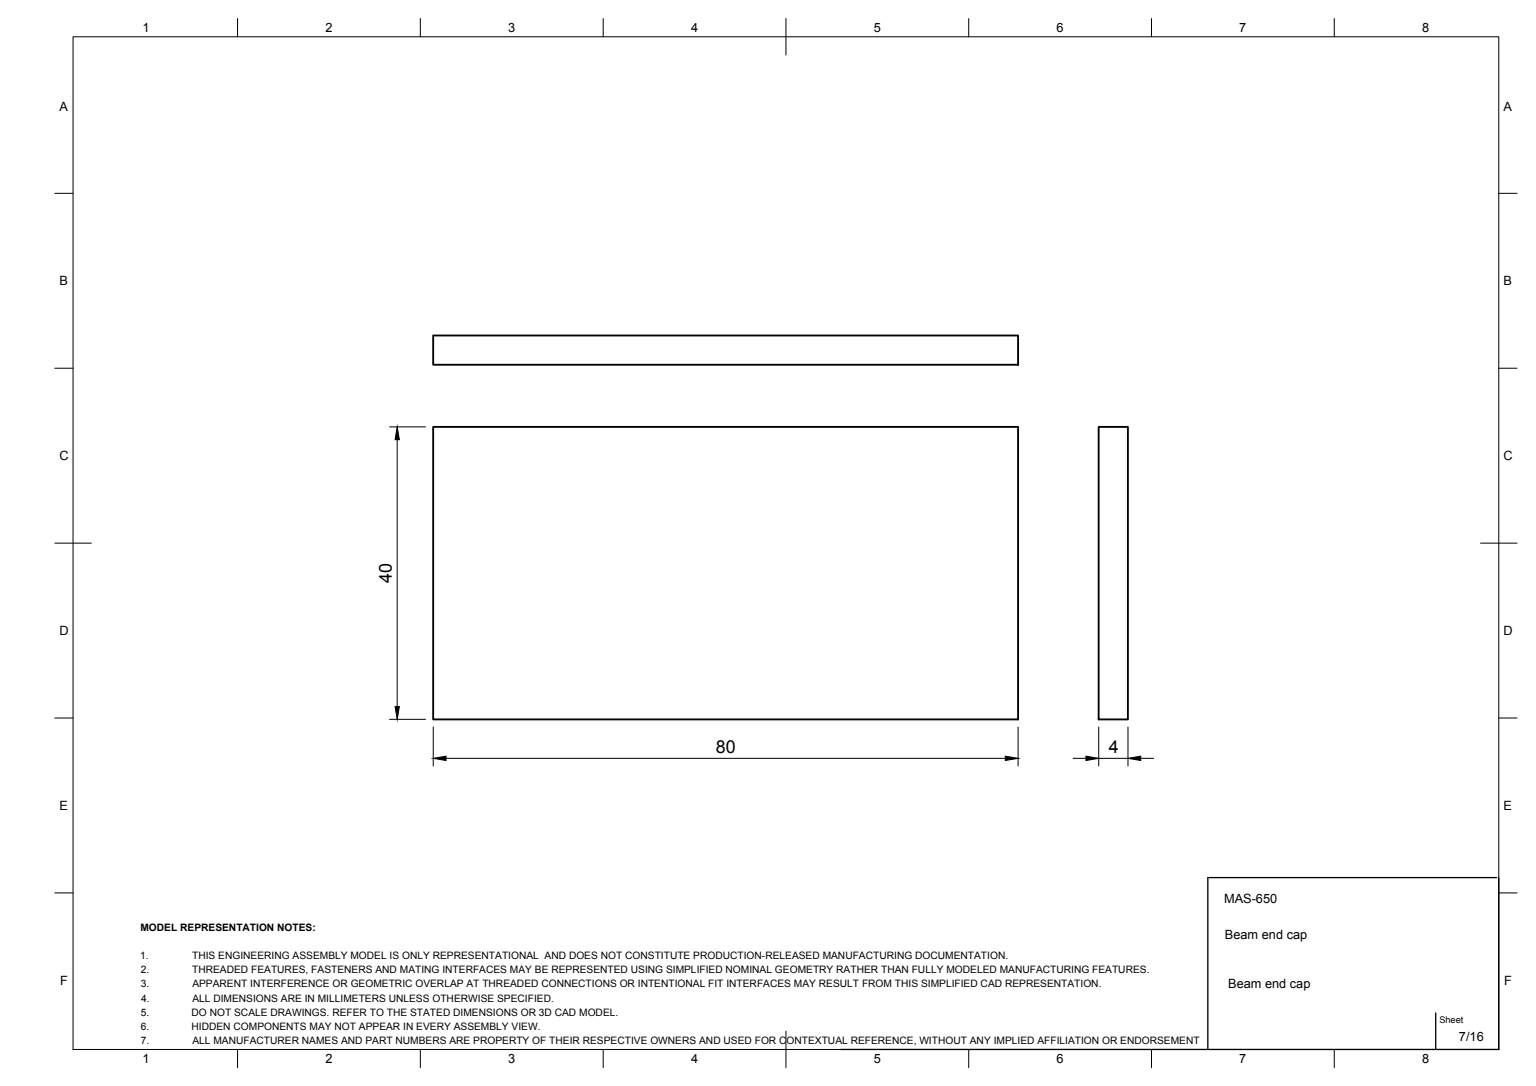
ISO-10303-21;
HEADER;
/* Generated by software containing ST-Developer
 * from STEP Tools, Inc. (www.steptools.com) 
 */

FILE_DESCRIPTION(
/* description */ ('Independent manual traversing gantry with native reusable aluminum pr
ofiles,180mm captured carriage travel, four bronze-bushed rollers, lin
ked ideal rolling motion, bonded acetal lateral guides, positive welde
d end stops and fully retained axle stacks. Editable native profile cu
t lengths220/400mm. Tool attachments viaM6 bridge-plate taps; mounted 
tool outside assembly. Welds, anchors, adhesives, fits, traction, load
/speed/structural/life ratings unassigned.'),
/* implementation_level */ '2;1');

FILE_NAME(
/* name */ 'Beam end cap.step',
/* time_stamp */ '2026-11-09T20:04:38-08:00',
/* author */ (''),
/* organization */ (''),
/* preprocessor_version */ 'ST-DEVELOPER v20.2',
/* originating_system */ 'Autodesk Translation Framework v15.17.0.0',
/* authorisation */ '');

FILE_SCHEMA (('AUTOMOTIVE_DESIGN { 1 0 10303 214 3 1 1 }'));
ENDSEC;

DATA;
#10=MECHANICAL_DESIGN_GEOMETRIC_PRESENTATION_REPRESENTATION('',(#475),#13231);
#443=SHAPE_REPRESENTATION_RELATIONSHIP('SRR','None',#13332,#459);
#459=ADVANCED_BREP_SHAPE_REPRESENTATION('',(#491),#13219);
#475=STYLED_ITEM('',(#13421),#491);
#491=MANIFOLD_SOLID_BREP('Body1',#4155);
#584=PLANE('',#4454);
#585=PLANE('',#4455);
#586=PLANE('',#4456);
#587=PLANE('',#4457);
#588=PLANE('',#4458);
#589=PLANE('',#4459);
#689=FACE_OUTER_BOUND('',#930,.T.);
#690=FACE_OUTER_BOUND('',#931,.T.);
#691=FACE_OUTER_BOUND('',#932,.T.);
#692=FACE_OUTER_BOUND('',#933,.T.);
#693=FACE_OUTER_BOUND('',#934,.T.);
#694=FACE_OUTER_BOUND('',#935,.T.);
#930=EDGE_LOOP('',(#2970,#2971,#2972,#2973));
#931=EDGE_LOOP('',(#2974,#2975,#2976,#2977));
#932=EDGE_LOOP('',(#2978,#2979,#2980,#2981));
#933=EDGE_LOOP('',(#2982,#2983,#2984,#2985));
#934=EDGE_LOOP('',(#2986,#2987,#2988,#2989));
#935=EDGE_LOOP('',(#2990,#2991,#2992,#2993));
#1220=LINE('',#6084,#1482);
#1221=LINE('',#6086,#1483);
#1222=LINE('',#6088,#1484);
#1223=LINE('',#6089,#1485);
#1224=LINE('',#6092,#1486);
#1225=LINE('',#6094,#1487);
#1226=LINE('',#6095,#1488);
#1227=LINE('',#6098,#1489);
#1228=LINE('',#6100,#1490);
#1229=LINE('',#6101,#1491);
#1230=LINE('',#6103,#1492);
#1231=LINE('',#6104,#1493);
#1482=VECTOR('',#5053,10.);
#1483=VECTOR('',#5054,10.);
#1484=VECTOR('',#5055,10.);
#1485=VECTOR('',#5056,10.);
#1486=VECTOR('',#5059,10.);
#1487=VECTOR('',#5060,10.);
#1488=VECTOR('',#5061,10.);
#1489=VECTOR('',#5064,10.);
#1490=VECTOR('',#5065,10.);
#1491=VECTOR('',#5066,10.);
#1492=VECTOR('',#5069,10.);
#1493=VECTOR('',#5070,10.);
#1848=VERTEX_POINT('',#6082);
#1849=VERTEX_POINT('',#6083);
#1850=VERTEX_POINT('',#6085);
#1851=VERTEX_POINT('',#6087);
#1852=VERTEX_POINT('',#6091);
#1853=VERTEX_POINT('',#6093);
#1854=VERTEX_POINT('',#6097);
#1855=VERTEX_POINT('',#6099);
#2268=EDGE_CURVE('',#1848,#1849,#1220,.T.);
#2269=EDGE_CURVE('',#1849,#1850,#1221,.T.);
#2270=EDGE_CURVE('',#1851,#1850,#1222,.T.);
#2271=EDGE_CURVE('',#1848,#1851,#1223,.T.);
#2272=EDGE_CURVE('',#1852,#1848,#1224,.T.);
#2273=EDGE_CURVE('',#1853,#1851,#1225,.T.);
#2274=EDGE_CURVE('',#1852,#1853,#1226,.T.);
#2275=EDGE_CURVE('',#1854,#1852,#1227,.T.);
#2276=EDGE_CURVE('',#1855,#1853,#1228,.T.);
#2277=EDGE_CURVE('',#1854,#1855,#1229,.T.);
#2278=EDGE_CURVE('',#1849,#1854,#1230,.T.);
#2279=EDGE_CURVE('',#1850,#1855,#1231,.T.);
#2970=ORIENTED_EDGE('',*,*,#2268,.T.);
#2971=ORIENTED_EDGE('',*,*,#2269,.T.);
#2972=ORIENTED_EDGE('',*,*,#2270,.F.);
#2973=ORIENTED_EDGE('',*,*,#2271,.F.);
#2974=ORIENTED_EDGE('',*,*,#2272,.T.);
#2975=ORIENTED_EDGE('',*,*,#2271,.T.);
#2976=ORIENTED_EDGE('',*,*,#2273,.F.);
#2977=ORIENTED_EDGE('',*,*,#2274,.F.);
#2978=ORIENTED_EDGE('',*,*,#2275,.T.);
#2979=ORIENTED_EDGE('',*,*,#2274,.T.);
#2980=ORIENTED_EDGE('',*,*,#2276,.F.);
#2981=ORIENTED_EDGE('',*,*,#2277,.F.);
#2982=ORIENTED_EDGE('',*,*,#2278,.T.);
#2983=ORIENTED_EDGE('',*,*,#2277,.T.);
#2984=ORIENTED_EDGE('',*,*,#2279,.F.);
#2985=ORIENTED_EDGE('',*,*,#2269,.F.);
#2986=ORIENTED_EDGE('',*,*,#2279,.T.);
#2987=ORIENTED_EDGE('',*,*,#2276,.T.);
#2988=ORIENTED_EDGE('',*,*,#2273,.T.);
#2989=ORIENTED_EDGE('',*,*,#2270,.T.);
#2990=ORIENTED_EDGE('',*,*,#2278,.F.);
#2991=ORIENTED_EDGE('',*,*,#2268,.F.);
#2992=ORIENTED_EDGE('',*,*,#2272,.F.);
#2993=ORIENTED_EDGE('',*,*,#2275,.F.);
#3986=ADVANCED_FACE('',(#689),#584,.T.);
#3987=ADVANCED_FACE('',(#690),#585,.T.);
#3988=ADVANCED_FACE('',(#691),#586,.T.);
#3989=ADVANCED_FACE('',(#692),#587,.T.);
#3990=ADVANCED_FACE('',(#693),#588,.T.);
#3991=ADVANCED_FACE('',(#694),#589,.F.);
#4155=CLOSED_SHELL('',(#3986,#3987,#3988,#3989,#3990,#3991));
#4453=AXIS2_PLACEMENT_3D('',#6080,#5049,#5050);
#4454=AXIS2_PLACEMENT_3D('',#6081,#5051,#5052);
#4455=AXIS2_PLACEMENT_3D('',#6090,#5057,#5058);
#4456=AXIS2_PLACEMENT_3D('',#6096,#5062,#5063);
#4457=AXIS2_PLACEMENT_3D('',#6102,#5067,#5068);
#4458=AXIS2_PLACEMENT_3D('',#6105,#5071,#5072);
#4459=AXIS2_PLACEMENT_3D('',#6106,#5073,#5074);
#5049=DIRECTION('axis',(0.,0.,1.));
#5050=DIRECTION('refdir',(1.,0.,0.));
#5051=DIRECTION('center_axis',(0.,1.,0.));
#5052=DIRECTION('ref_axis',(-1.,0.,0.));
#5053=DIRECTION('',(-1.,0.,0.));
#5054=DIRECTION('',(0.,0.,1.));
#5055=DIRECTION('',(-1.,0.,0.));
#5056=DIRECTION('',(0.,0.,1.));
#5057=DIRECTION('center_axis',(1.,0.,0.));
#5058=DIRECTION('ref_axis',(0.,1.,0.));
#5059=DIRECTION('',(0.,1.,0.));
#5060=DIRECTION('',(0.,1.,0.));
#5061=DIRECTION('',(0.,0.,1.));
#5062=DIRECTION('center_axis',(0.,-1.,0.));
#5063=DIRECTION('ref_axis',(1.,0.,0.));
#5064=DIRECTION('',(1.,0.,0.));
#5065=DIRECTION('',(1.,0.,0.));
#5066=DIRECTION('',(0.,0.,1.));
#5067=DIRECTION('center_axis',(-1.,0.,0.));
#5068=DIRECTION('ref_axis',(0.,-1.,0.));
#5069=DIRECTION('',(0.,-1.,0.));
#5070=DIRECTION('',(0.,-1.,0.));
#5071=DIRECTION('center_axis',(0.,0.,1.));
#5072=DIRECTION('ref_axis',(1.,0.,0.));
#5073=DIRECTION('center_axis',(0.,0.,1.));
#5074=DIRECTION('ref_axis',(1.,0.,0.));
#6080=CARTESIAN_POINT('',(0.,0.,0.));
#6081=CARTESIAN_POINT('Origin',(40.,20.,0.));
#6082=CARTESIAN_POINT('',(40.,20.,0.));
#6083=CARTESIAN_POINT('',(-40.,20.,0.));
#6084=CARTESIAN_POINT('',(40.,20.,0.));
#6085=CARTESIAN_POINT('',(-40.,20.,4.));
#6086=CARTESIAN_POINT('',(-40.,20.,0.));
#6087=CARTESIAN_POINT('',(40.,20.,4.));
#6088=CARTESIAN_POINT('',(40.,20.,4.));
#6089=CARTESIAN_POINT('',(40.,20.,0.));
#6090=CARTESIAN_POINT('Origin',(40.,-20.,0.));
#6091=CARTESIAN_POINT('',(40.,-20.,0.));
#6092=CARTESIAN_POINT('',(40.,-20.,0.));
#6093=CARTESIAN_POINT('',(40.,-20.,4.));
#6094=CARTESIAN_POINT('',(40.,-20.,4.));
#6095=CARTESIAN_POINT('',(40.,-20.,0.));
#6096=CARTESIAN_POINT('Origin',(-40.,-20.,0.));
#6097=CARTESIAN_POINT('',(-40.,-20.,0.));
#6098=CARTESIAN_POINT('',(-40.,-20.,0.));
#6099=CARTESIAN_POINT('',(-40.,-20.,4.));
#6100=CARTESIAN_POINT('',(-40.,-20.,4.));
#6101=CARTESIAN_POINT('',(-40.,-20.,0.));
#6102=CARTESIAN_POINT('Origin',(-40.,20.,0.));
#6103=CARTESIAN_POINT('',(-40.,20.,0.));
#6104=CARTESIAN_POINT('',(-40.,20.,4.));
#6105=CARTESIAN_POINT('Origin',(0.,0.,4.));
#6106=CARTESIAN_POINT('Origin',(0.,0.,0.));
#13201=UNCERTAINTY_MEASURE_WITH_UNIT(LENGTH_MEASURE(0.01),#13232,
'DISTANCE_ACCURACY_VALUE',
'Maximum model space distance between geometric entities at asserted c
onnectivities');
#13213=UNCERTAINTY_MEASURE_WITH_UNIT(LENGTH_MEASURE(0.01),#13232,
'DISTANCE_ACCURACY_VALUE',
'Maximum model space distance between geometric entities at asserted c
onnectivities');
#13219=(
GEOMETRIC_REPRESENTATION_CONTEXT(3)
GLOBAL_UNCERTAINTY_ASSIGNED_CONTEXT((#13201))
GLOBAL_UNIT_ASSIGNED_CONTEXT((#13232,#13234,#13235))
REPRESENTATION_CONTEXT('','3D')
);
#13231=(
GEOMETRIC_REPRESENTATION_CONTEXT(3)
GLOBAL_UNCERTAINTY_ASSIGNED_CONTEXT((#13213))
GLOBAL_UNIT_ASSIGNED_CONTEXT((#13232,#13234,#13235))
REPRESENTATION_CONTEXT('','3D')
);
#13232=(
LENGTH_UNIT()
NAMED_UNIT(*)
SI_UNIT(.MILLI.,.METRE.)
);
#13234=(
NAMED_UNIT(*)
PLANE_ANGLE_UNIT()
SI_UNIT($,.RADIAN.)
);
#13235=(
NAMED_UNIT(*)
SI_UNIT($,.STERADIAN.)
SOLID_ANGLE_UNIT()
);
#13241=SHAPE_DEFINITION_REPRESENTATION(#13258,#13332);
#13258=PRODUCT_DEFINITION_SHAPE('',$,#13350);
#13332=SHAPE_REPRESENTATION('',(#4453),#13219);
#13344=PRODUCT_DEFINITION_CONTEXT('part definition',#13397,'design');
#13350=PRODUCT_DEFINITION('Beam end cap','Beam end cap',#13367,#13344);
#13367=PRODUCT_DEFINITION_FORMATION('',$,#13404);
#13397=APPLICATION_CONTEXT(
'Core Data for Automotive Mechanical Design Process');
#13398=PRODUCT_CONTEXT('part definition',#13397,'mechanical');
#13404=PRODUCT('Beam end cap','Beam end cap',$,(#13398));
#13421=PRESENTATION_STYLE_ASSIGNMENT((#13435));
#13435=SURFACE_STYLE_USAGE(.BOTH.,#13449);
#13449=SURFACE_SIDE_STYLE('',(#13463));
#13463=SURFACE_STYLE_FILL_AREA(#13477);
#13477=FILL_AREA_STYLE('Light gray',(#13491));
#13491=FILL_AREA_STYLE_COLOUR('Light gray',#13505);
#13505=COLOUR_RGB('Light gray',0.725490196078431,0.752941176470588,0.792156862745098);
ENDSEC;
END-ISO-10303-21;
